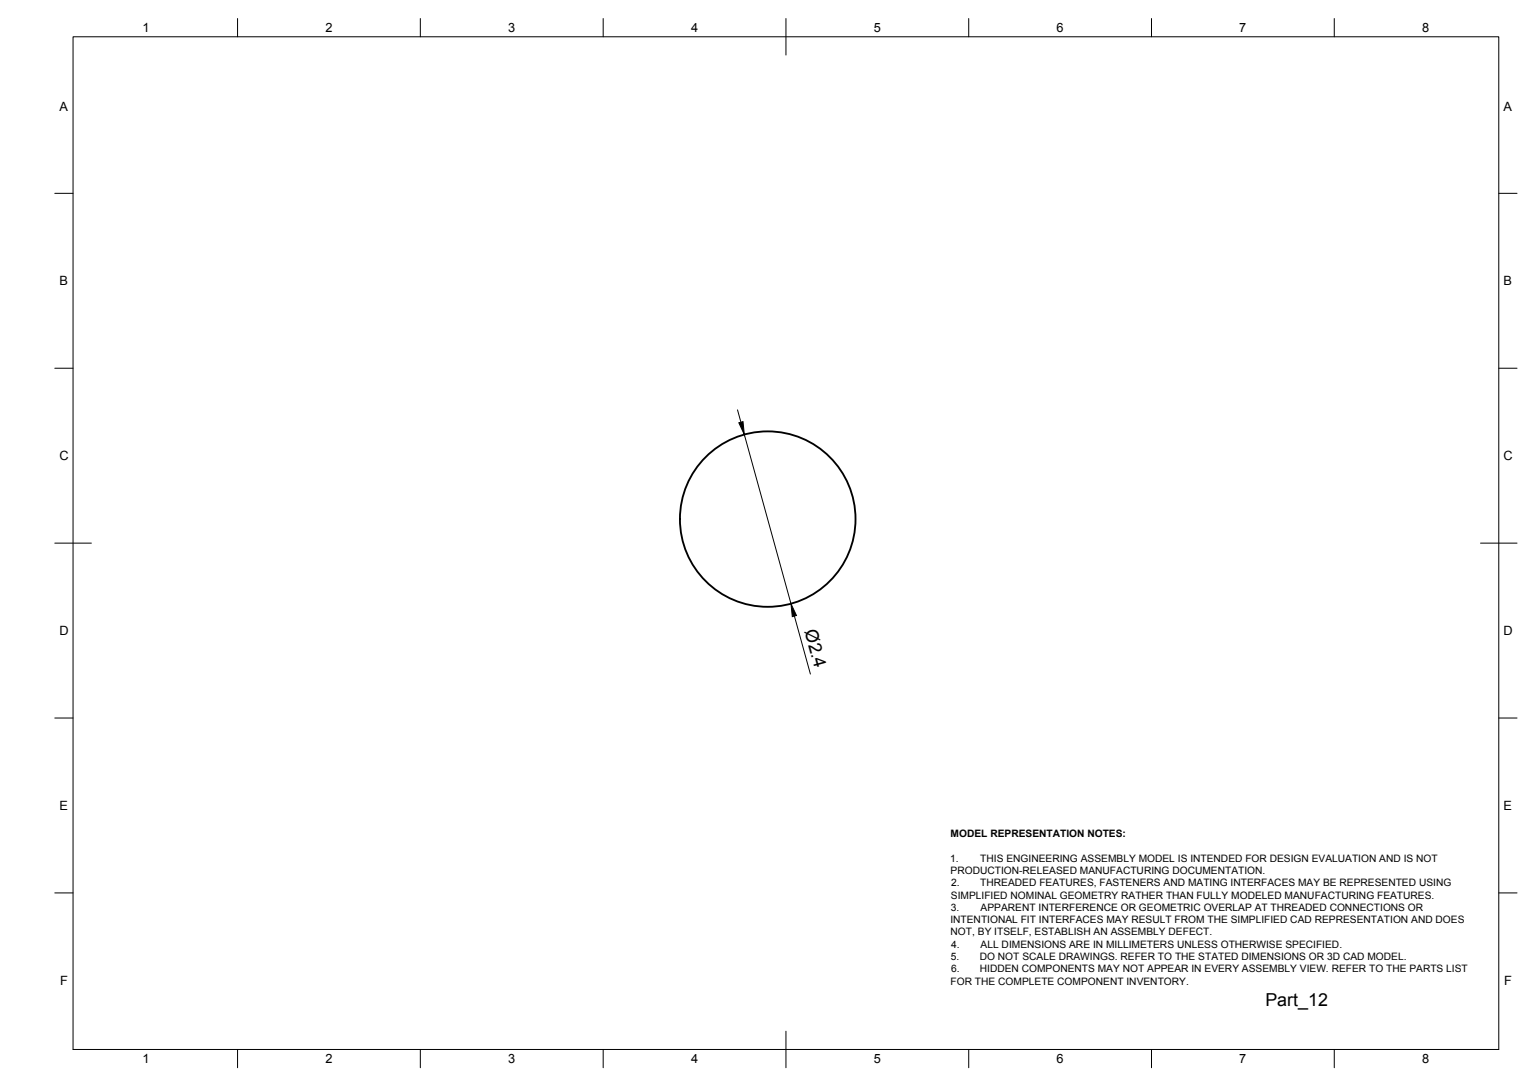
ISO-10303-21;
HEADER;
/* Generated by software containing ST-Developer
 * from STEP Tools, Inc. (www.steptools.com) 
 */

FILE_DESCRIPTION(
/* description */ ('STEP AP242 Edition 2'),
/* implementation_level */ '2;1');

FILE_NAME(
/* name */ 'Part_12.step',
/* time_stamp */ '2026-10-06T10:11:12-07:00',
/* author */ (''),
/* organization */ (''),
/* preprocessor_version */ 'ST-DEVELOPER v20.2',
/* originating_system */ 'Autodesk Translation Framework v15.15.0.0',
/* authorisation */ '');

FILE_SCHEMA (('AUTOMOTIVE_DESIGN { 1 0 10303 214 3 1 1 }'));
ENDSEC;

DATA;
#10=MECHANICAL_DESIGN_GEOMETRIC_PRESENTATION_REPRESENTATION('',(#1785),#54580);
#142=SPHERICAL_SURFACE('',#18518,0.0012);
#1745=SHAPE_REPRESENTATION_RELATIONSHIP('SRR','None',#54632,#1759);
#1759=ADVANCED_BREP_SHAPE_REPRESENTATION('',(#1803),#54568);
#1785=STYLED_ITEM('',(#54713),#1803);
#1803=MANIFOLD_SOLID_BREP('Body1',#17668);
#3780=FACE_OUTER_BOUND('',#4791,.T.);
#4791=EDGE_LOOP('',(#12415,#12416));
#6070=CIRCLE('',#18519,0.0012);
#6970=VERTEX_POINT('',#25841);
#6971=VERTEX_POINT('',#25842);
#8999=EDGE_CURVE('',#6970,#6971,#6070,.T.);
#12415=ORIENTED_EDGE('',*,*,#8999,.F.);
#12416=ORIENTED_EDGE('',*,*,#8999,.T.);
#16896=ADVANCED_FACE('',(#3780),#142,.T.);
#17668=CLOSED_SHELL('',(#16896));
#18517=AXIS2_PLACEMENT_3D('',#25839,#21167,#21168);
#18518=AXIS2_PLACEMENT_3D('',#25840,#21169,#21170);
#18519=AXIS2_PLACEMENT_3D('',#25843,#21171,#21172);
#21167=DIRECTION('axis',(0.,0.,1.));
#21168=DIRECTION('refdir',(1.,0.,0.));
#21169=DIRECTION('center_axis',(0.,1.,0.));
#21170=DIRECTION('ref_axis',(1.,0.,0.));
#21171=DIRECTION('center_axis',(1.22464679914735E-16,1.97778073784536E-32,
1.));
#21172=DIRECTION('ref_axis',(-1.,0.,1.22464679914735E-16));
#25839=CARTESIAN_POINT('',(0.,0.,0.));
#25840=CARTESIAN_POINT('Origin',(-0.00333123939879042,-0.00899999999999701,
0.));
#25841=CARTESIAN_POINT('',(-0.00333123939879042,-0.00779999999999701,-1.47348101581732E-35));
#25842=CARTESIAN_POINT('',(-0.00333123939879042,-0.010199999999997,0.));
#25843=CARTESIAN_POINT('Origin',(-0.00333123939879042,-0.00899999999999701,
0.));
#54552=UNCERTAINTY_MEASURE_WITH_UNIT(LENGTH_MEASURE(1.E-5),#54581,
'DISTANCE_ACCURACY_VALUE',
'Maximum model space distance between geometric entities at asserted c
onnectivities');
#54564=UNCERTAINTY_MEASURE_WITH_UNIT(LENGTH_MEASURE(1.E-5),#54581,
'DISTANCE_ACCURACY_VALUE',
'Maximum model space distance between geometric entities at asserted c
onnectivities');
#54568=(
GEOMETRIC_REPRESENTATION_CONTEXT(3)
GLOBAL_UNCERTAINTY_ASSIGNED_CONTEXT((#54552))
GLOBAL_UNIT_ASSIGNED_CONTEXT((#54581,#54582,#54583))
REPRESENTATION_CONTEXT('','3D')
);
#54580=(
GEOMETRIC_REPRESENTATION_CONTEXT(3)
GLOBAL_UNCERTAINTY_ASSIGNED_CONTEXT((#54564))
GLOBAL_UNIT_ASSIGNED_CONTEXT((#54581,#54582,#54583))
REPRESENTATION_CONTEXT('','3D')
);
#54581=(
LENGTH_UNIT()
NAMED_UNIT(*)
SI_UNIT($,.METRE.)
);
#54582=(
NAMED_UNIT(*)
PLANE_ANGLE_UNIT()
SI_UNIT($,.RADIAN.)
);
#54583=(
NAMED_UNIT(*)
SI_UNIT($,.STERADIAN.)
SOLID_ANGLE_UNIT()
);
#54587=SHAPE_DEFINITION_REPRESENTATION(#54602,#54632);
#54602=PRODUCT_DEFINITION_SHAPE('',$,#54648);
#54632=SHAPE_REPRESENTATION('',(#18517),#54568);
#54644=PRODUCT_DEFINITION_CONTEXT('part definition',#54691,'design');
#54648=PRODUCT_DEFINITION('Part_12','Part_12',#54663,#54644);
#54663=PRODUCT_DEFINITION_FORMATION('',$,#54696);
#54691=APPLICATION_CONTEXT(
'Core Data for Automotive Mechanical Design Process');
#54692=PRODUCT_CONTEXT('part definition',#54691,'mechanical');
#54696=PRODUCT('Part_12','Part_12','Part 1',(#54692));
#54713=PRESENTATION_STYLE_ASSIGNMENT((#54723));
#54723=SURFACE_STYLE_USAGE(.BOTH.,#54733);
#54733=SURFACE_SIDE_STYLE('',(#54743));
#54743=SURFACE_STYLE_FILL_AREA(#54753);
#54753=FILL_AREA_STYLE('Opaque(163,170,173)',(#54763));
#54763=FILL_AREA_STYLE_COLOUR('Opaque(163,170,173)',#54773);
#54773=COLOUR_RGB('Opaque(163,170,173)', 0.31764706, 0.68627451, 0.89019608);
ENDSEC;
END-ISO-10303-21;
